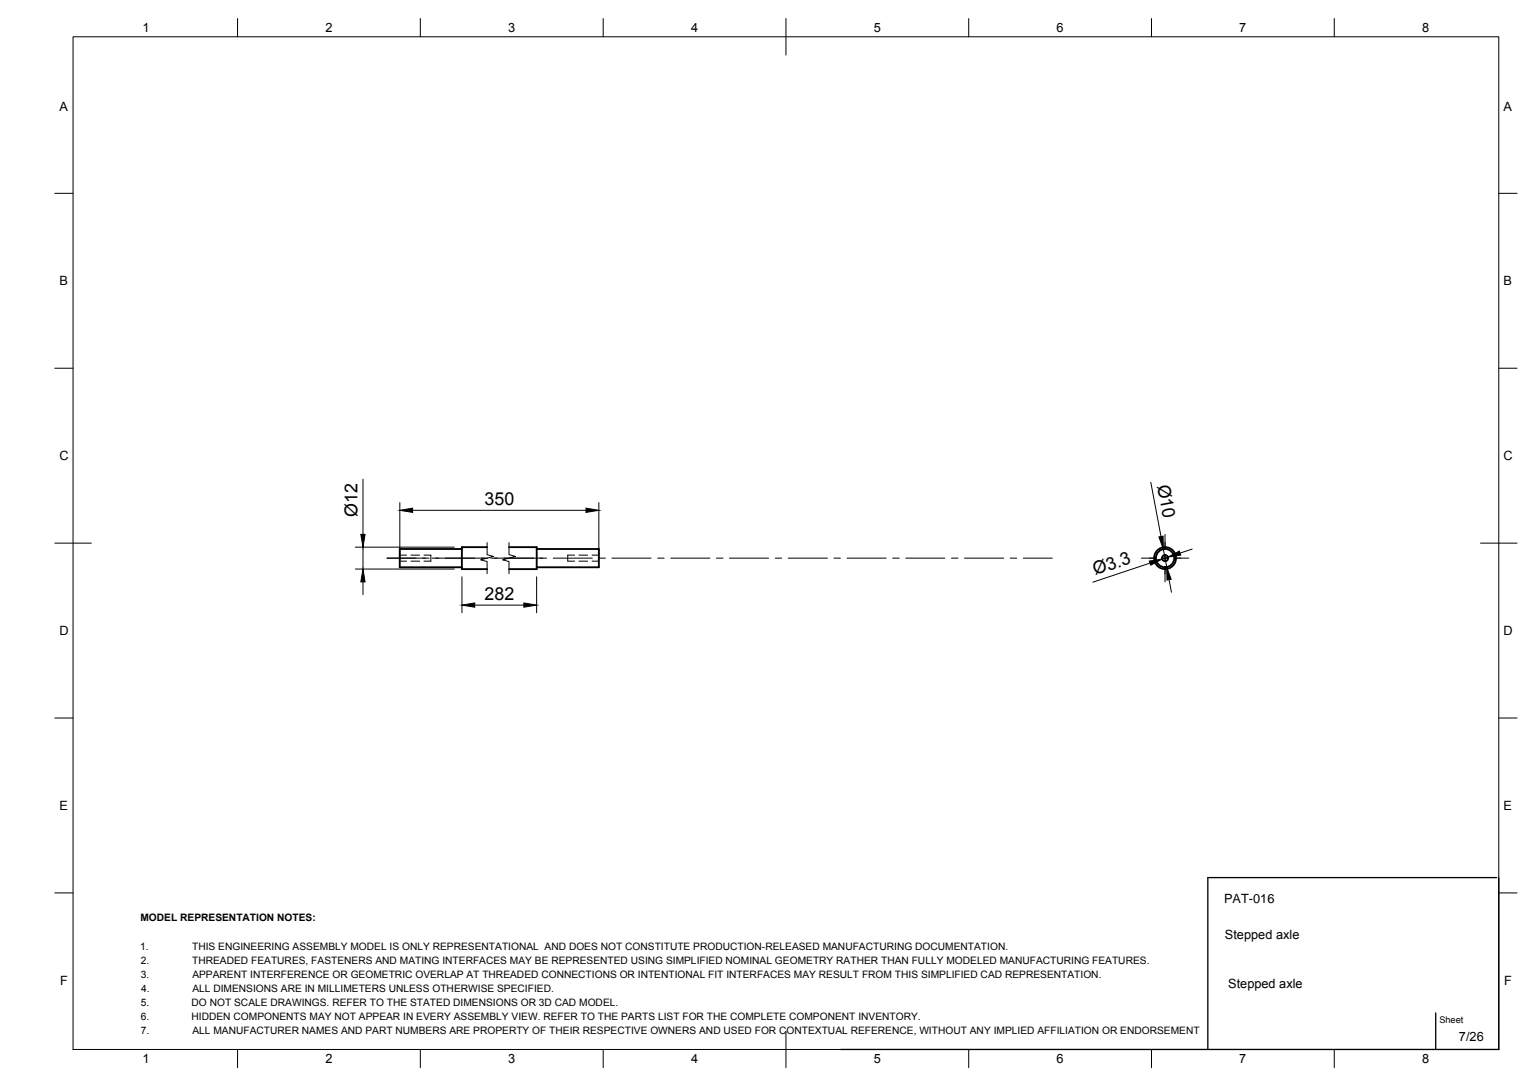
ISO-10303-21;
HEADER;
/* Generated by software containing ST-Developer
 * from STEP Tools, Inc. (www.steptools.com) 
 */

FILE_DESCRIPTION(
/* description */ ('Bracket-mounted idler roller'),
/* implementation_level */ '2;1');

FILE_NAME(
/* name */ 'Stepped axle.step',
/* time_stamp */ '2026-10-28T03:26:42-07:00',
/* author */ (''),
/* organization */ (''),
/* preprocessor_version */ 'ST-DEVELOPER v20.2',
/* originating_system */ 'Autodesk Translation Framework v15.17.0.0',
/* authorisation */ '');

FILE_SCHEMA (('AUTOMOTIVE_DESIGN { 1 0 10303 214 3 1 1 }'));
ENDSEC;

DATA;
#10=MECHANICAL_DESIGN_GEOMETRIC_PRESENTATION_REPRESENTATION('',(#282),#6241);
#240=SHAPE_REPRESENTATION_RELATIONSHIP('SRR','None',#6344,#261);
#261=ADVANCED_BREP_SHAPE_REPRESENTATION('',(#311),#6220);
#282=STYLED_ITEM('',(#6538),#311);
#311=MANIFOLD_SOLID_BREP('Body1',#3184);
#350=FACE_BOUND('',#754,.T.);
#351=FACE_BOUND('',#756,.T.);
#352=FACE_BOUND('',#761,.T.);
#353=FACE_BOUND('',#763,.T.);
#439=PLANE('',#3493);
#440=PLANE('',#3497);
#441=PLANE('',#3498);
#442=PLANE('',#3501);
#443=PLANE('',#3509);
#444=PLANE('',#3510);
#544=FACE_OUTER_BOUND('',#749,.T.);
#545=FACE_OUTER_BOUND('',#750,.T.);
#546=FACE_OUTER_BOUND('',#751,.T.);
#547=FACE_OUTER_BOUND('',#752,.T.);
#548=FACE_OUTER_BOUND('',#753,.T.);
#549=FACE_OUTER_BOUND('',#755,.T.);
#550=FACE_OUTER_BOUND('',#757,.T.);
#551=FACE_OUTER_BOUND('',#758,.T.);
#552=FACE_OUTER_BOUND('',#759,.T.);
#553=FACE_OUTER_BOUND('',#760,.T.);
#554=FACE_OUTER_BOUND('',#762,.T.);
#749=EDGE_LOOP('',(#2298,#2299,#2300,#2301));
#750=EDGE_LOOP('',(#2302));
#751=EDGE_LOOP('',(#2303,#2304,#2305,#2306));
#752=EDGE_LOOP('',(#2307));
#753=EDGE_LOOP('',(#2308));
#754=EDGE_LOOP('',(#2309));
#755=EDGE_LOOP('',(#2310));
#756=EDGE_LOOP('',(#2311));
#757=EDGE_LOOP('',(#2312,#2313,#2314,#2315));
#758=EDGE_LOOP('',(#2316,#2317,#2318,#2319));
#759=EDGE_LOOP('',(#2320,#2321,#2322,#2323));
#760=EDGE_LOOP('',(#2324));
#761=EDGE_LOOP('',(#2325));
#762=EDGE_LOOP('',(#2326));
#763=EDGE_LOOP('',(#2327));
#1033=LINE('',#5097,#1215);
#1034=LINE('',#5104,#1216);
#1035=LINE('',#5118,#1217);
#1036=LINE('',#5121,#1218);
#1037=LINE('',#5126,#1219);
#1215=VECTOR('',#4034,0.165);
#1216=VECTOR('',#4043,0.165);
#1217=VECTOR('',#4062,0.6);
#1218=VECTOR('',#4065,0.5);
#1219=VECTOR('',#4072,0.5);
#1355=CIRCLE('',#3491,0.165);
#1356=CIRCLE('',#3492,0.165);
#1357=CIRCLE('',#3495,0.165);
#1358=CIRCLE('',#3496,0.165);
#1359=CIRCLE('',#3499,0.6);
#1360=CIRCLE('',#3500,0.5);
#1361=CIRCLE('',#3502,0.6);
#1362=CIRCLE('',#3503,0.5);
#1363=CIRCLE('',#3506,0.5);
#1364=CIRCLE('',#3508,0.5);
#1568=VERTEX_POINT('',#5094);
#1569=VERTEX_POINT('',#5096);
#1570=VERTEX_POINT('',#5101);
#1571=VERTEX_POINT('',#5103);
#1572=VERTEX_POINT('',#5108);
#1573=VERTEX_POINT('',#5110);
#1574=VERTEX_POINT('',#5113);
#1575=VERTEX_POINT('',#5115);
#1576=VERTEX_POINT('',#5120);
#1577=VERTEX_POINT('',#5124);
#1851=EDGE_CURVE('',#1568,#1568,#1355,.T.);
#1852=EDGE_CURVE('',#1568,#1569,#1033,.T.);
#1853=EDGE_CURVE('',#1569,#1569,#1356,.T.);
#1854=EDGE_CURVE('',#1570,#1570,#1357,.T.);
#1855=EDGE_CURVE('',#1570,#1571,#1034,.T.);
#1856=EDGE_CURVE('',#1571,#1571,#1358,.T.);
#1857=EDGE_CURVE('',#1572,#1572,#1359,.T.);
#1858=EDGE_CURVE('',#1573,#1573,#1360,.T.);
#1859=EDGE_CURVE('',#1574,#1574,#1361,.T.);
#1860=EDGE_CURVE('',#1575,#1575,#1362,.T.);
#1861=EDGE_CURVE('',#1572,#1574,#1035,.T.);
#1862=EDGE_CURVE('',#1575,#1576,#1036,.T.);
#1863=EDGE_CURVE('',#1576,#1576,#1363,.T.);
#1864=EDGE_CURVE('',#1577,#1577,#1364,.T.);
#1865=EDGE_CURVE('',#1577,#1573,#1037,.T.);
#2298=ORIENTED_EDGE('',*,*,#1851,.F.);
#2299=ORIENTED_EDGE('',*,*,#1852,.T.);
#2300=ORIENTED_EDGE('',*,*,#1853,.F.);
#2301=ORIENTED_EDGE('',*,*,#1852,.F.);
#2302=ORIENTED_EDGE('',*,*,#1851,.T.);
#2303=ORIENTED_EDGE('',*,*,#1854,.F.);
#2304=ORIENTED_EDGE('',*,*,#1855,.T.);
#2305=ORIENTED_EDGE('',*,*,#1856,.T.);
#2306=ORIENTED_EDGE('',*,*,#1855,.F.);
#2307=ORIENTED_EDGE('',*,*,#1856,.F.);
#2308=ORIENTED_EDGE('',*,*,#1857,.T.);
#2309=ORIENTED_EDGE('',*,*,#1858,.F.);
#2310=ORIENTED_EDGE('',*,*,#1859,.F.);
#2311=ORIENTED_EDGE('',*,*,#1860,.F.);
#2312=ORIENTED_EDGE('',*,*,#1857,.F.);
#2313=ORIENTED_EDGE('',*,*,#1861,.T.);
#2314=ORIENTED_EDGE('',*,*,#1859,.T.);
#2315=ORIENTED_EDGE('',*,*,#1861,.F.);
#2316=ORIENTED_EDGE('',*,*,#1860,.T.);
#2317=ORIENTED_EDGE('',*,*,#1862,.T.);
#2318=ORIENTED_EDGE('',*,*,#1863,.T.);
#2319=ORIENTED_EDGE('',*,*,#1862,.F.);
#2320=ORIENTED_EDGE('',*,*,#1864,.F.);
#2321=ORIENTED_EDGE('',*,*,#1865,.T.);
#2322=ORIENTED_EDGE('',*,*,#1858,.T.);
#2323=ORIENTED_EDGE('',*,*,#1865,.F.);
#2324=ORIENTED_EDGE('',*,*,#1864,.T.);
#2325=ORIENTED_EDGE('',*,*,#1853,.T.);
#2326=ORIENTED_EDGE('',*,*,#1863,.F.);
#2327=ORIENTED_EDGE('',*,*,#1854,.T.);
#2934=CYLINDRICAL_SURFACE('',#3490,0.165);
#2935=CYLINDRICAL_SURFACE('',#3494,0.165);
#2936=CYLINDRICAL_SURFACE('',#3504,0.6);
#2937=CYLINDRICAL_SURFACE('',#3505,0.5);
#2938=CYLINDRICAL_SURFACE('',#3507,0.5);
#3019=ADVANCED_FACE('',(#544),#2934,.F.);
#3020=ADVANCED_FACE('',(#545),#439,.T.);
#3021=ADVANCED_FACE('',(#546),#2935,.F.);
#3022=ADVANCED_FACE('',(#547),#440,.F.);
#3023=ADVANCED_FACE('',(#548,#350),#441,.T.);
#3024=ADVANCED_FACE('',(#549,#351),#442,.F.);
#3025=ADVANCED_FACE('',(#550),#2936,.T.);
#3026=ADVANCED_FACE('',(#551),#2937,.T.);
#3027=ADVANCED_FACE('',(#552),#2938,.T.);
#3028=ADVANCED_FACE('',(#553,#352),#443,.T.);
#3029=ADVANCED_FACE('',(#554,#353),#444,.F.);
#3184=CLOSED_SHELL('',(#3019,#3020,#3021,#3022,#3023,#3024,#3025,#3026,
#3027,#3028,#3029));
#3489=AXIS2_PLACEMENT_3D('',#5092,#4028,#4029);
#3490=AXIS2_PLACEMENT_3D('',#5093,#4030,#4031);
#3491=AXIS2_PLACEMENT_3D('',#5095,#4032,#4033);
#3492=AXIS2_PLACEMENT_3D('',#5098,#4035,#4036);
#3493=AXIS2_PLACEMENT_3D('',#5099,#4037,#4038);
#3494=AXIS2_PLACEMENT_3D('',#5100,#4039,#4040);
#3495=AXIS2_PLACEMENT_3D('',#5102,#4041,#4042);
#3496=AXIS2_PLACEMENT_3D('',#5105,#4044,#4045);
#3497=AXIS2_PLACEMENT_3D('',#5106,#4046,#4047);
#3498=AXIS2_PLACEMENT_3D('',#5107,#4048,#4049);
#3499=AXIS2_PLACEMENT_3D('',#5109,#4050,#4051);
#3500=AXIS2_PLACEMENT_3D('',#5111,#4052,#4053);
#3501=AXIS2_PLACEMENT_3D('',#5112,#4054,#4055);
#3502=AXIS2_PLACEMENT_3D('',#5114,#4056,#4057);
#3503=AXIS2_PLACEMENT_3D('',#5116,#4058,#4059);
#3504=AXIS2_PLACEMENT_3D('',#5117,#4060,#4061);
#3505=AXIS2_PLACEMENT_3D('',#5119,#4063,#4064);
#3506=AXIS2_PLACEMENT_3D('',#5122,#4066,#4067);
#3507=AXIS2_PLACEMENT_3D('',#5123,#4068,#4069);
#3508=AXIS2_PLACEMENT_3D('',#5125,#4070,#4071);
#3509=AXIS2_PLACEMENT_3D('',#5127,#4073,#4074);
#3510=AXIS2_PLACEMENT_3D('',#5128,#4075,#4076);
#4028=DIRECTION('axis',(0.,0.,1.));
#4029=DIRECTION('refdir',(1.,0.,0.));
#4030=DIRECTION('center_axis',(0.,1.,0.));
#4031=DIRECTION('ref_axis',(1.,0.,0.));
#4032=DIRECTION('center_axis',(0.,1.,0.));
#4033=DIRECTION('ref_axis',(1.,0.,0.));
#4034=DIRECTION('',(0.,1.,0.));
#4035=DIRECTION('center_axis',(0.,-1.,0.));
#4036=DIRECTION('ref_axis',(1.,0.,0.));
#4037=DIRECTION('center_axis',(0.,1.,0.));
#4038=DIRECTION('ref_axis',(1.,0.,0.));
#4039=DIRECTION('center_axis',(0.,1.,0.));
#4040=DIRECTION('ref_axis',(1.,0.,0.));
#4041=DIRECTION('center_axis',(0.,1.,0.));
#4042=DIRECTION('ref_axis',(1.,0.,0.));
#4043=DIRECTION('',(0.,1.,0.));
#4044=DIRECTION('center_axis',(0.,1.,0.));
#4045=DIRECTION('ref_axis',(1.,0.,0.));
#4046=DIRECTION('center_axis',(0.,1.,0.));
#4047=DIRECTION('ref_axis',(1.,0.,0.));
#4048=DIRECTION('center_axis',(0.,1.,0.));
#4049=DIRECTION('ref_axis',(1.,0.,0.));
#4050=DIRECTION('center_axis',(0.,1.,0.));
#4051=DIRECTION('ref_axis',(1.,0.,0.));
#4052=DIRECTION('center_axis',(0.,1.,0.));
#4053=DIRECTION('ref_axis',(1.,0.,0.));
#4054=DIRECTION('center_axis',(0.,1.,0.));
#4055=DIRECTION('ref_axis',(1.,0.,0.));
#4056=DIRECTION('center_axis',(0.,1.,0.));
#4057=DIRECTION('ref_axis',(1.,0.,0.));
#4058=DIRECTION('center_axis',(0.,-1.,0.));
#4059=DIRECTION('ref_axis',(1.,0.,0.));
#4060=DIRECTION('center_axis',(0.,1.,0.));
#4061=DIRECTION('ref_axis',(1.,0.,0.));
#4062=DIRECTION('',(0.,-1.,0.));
#4063=DIRECTION('center_axis',(0.,1.,0.));
#4064=DIRECTION('ref_axis',(1.,0.,0.));
#4065=DIRECTION('',(0.,-1.,0.));
#4066=DIRECTION('center_axis',(0.,1.,0.));
#4067=DIRECTION('ref_axis',(1.,0.,0.));
#4068=DIRECTION('center_axis',(0.,1.,0.));
#4069=DIRECTION('ref_axis',(1.,0.,0.));
#4070=DIRECTION('center_axis',(0.,1.,0.));
#4071=DIRECTION('ref_axis',(1.,0.,0.));
#4072=DIRECTION('',(0.,-1.,0.));
#4073=DIRECTION('center_axis',(0.,1.,0.));
#4074=DIRECTION('ref_axis',(1.,0.,0.));
#4075=DIRECTION('center_axis',(0.,1.,0.));
#4076=DIRECTION('ref_axis',(1.,0.,0.));
#5092=CARTESIAN_POINT('',(0.,0.,0.));
#5093=CARTESIAN_POINT('Origin',(0.,30.8,4.5));
#5094=CARTESIAN_POINT('',(-0.165,30.8,4.5));
#5095=CARTESIAN_POINT('Origin',(0.,30.8,4.5));
#5096=CARTESIAN_POINT('',(-0.165,32.5,4.5));
#5097=CARTESIAN_POINT('',(-0.165,30.8,4.5));
#5098=CARTESIAN_POINT('Origin',(0.,32.5,4.5));
#5099=CARTESIAN_POINT('Origin',(0.,30.8,4.5));
#5100=CARTESIAN_POINT('Origin',(0.,-2.6,4.5));
#5101=CARTESIAN_POINT('',(-0.165,-2.5,4.5));
#5102=CARTESIAN_POINT('Origin',(0.,-2.5,4.5));
#5103=CARTESIAN_POINT('',(-0.165,-0.8,4.5));
#5104=CARTESIAN_POINT('',(-0.165,-2.6,4.5));
#5105=CARTESIAN_POINT('Origin',(0.,-0.8,4.5));
#5106=CARTESIAN_POINT('Origin',(0.,-0.8,4.5));
#5107=CARTESIAN_POINT('Origin',(0.,29.1,4.5));
#5108=CARTESIAN_POINT('',(-0.6,29.1,4.5));
#5109=CARTESIAN_POINT('Origin',(0.,29.1,4.5));
#5110=CARTESIAN_POINT('',(-0.5,29.1,4.5));
#5111=CARTESIAN_POINT('Origin',(0.,29.1,4.5));
#5112=CARTESIAN_POINT('Origin',(0.,0.9,4.5));
#5113=CARTESIAN_POINT('',(-0.6,0.9,4.5));
#5114=CARTESIAN_POINT('Origin',(0.,0.9,4.5));
#5115=CARTESIAN_POINT('',(-0.5,0.9,4.5));
#5116=CARTESIAN_POINT('Origin',(0.,0.9,4.5));
#5117=CARTESIAN_POINT('Origin',(0.,0.9,4.5));
#5118=CARTESIAN_POINT('',(-0.6,0.9,4.5));
#5119=CARTESIAN_POINT('Origin',(0.,-2.5,4.5));
#5120=CARTESIAN_POINT('',(-0.5,-2.5,4.5));
#5121=CARTESIAN_POINT('',(-0.5,-2.5,4.5));
#5122=CARTESIAN_POINT('Origin',(0.,-2.5,4.5));
#5123=CARTESIAN_POINT('Origin',(0.,-2.5,4.5));
#5124=CARTESIAN_POINT('',(-0.5,32.5,4.5));
#5125=CARTESIAN_POINT('Origin',(0.,32.5,4.5));
#5126=CARTESIAN_POINT('',(-0.5,-2.5,4.5));
#5127=CARTESIAN_POINT('Origin',(0.,32.5,4.5));
#5128=CARTESIAN_POINT('Origin',(0.,-2.5,4.5));
#6194=UNCERTAINTY_MEASURE_WITH_UNIT(LENGTH_MEASURE(0.001),#6242,
'DISTANCE_ACCURACY_VALUE',
'Maximum model space distance between geometric entities at asserted c
onnectivities');
#6215=UNCERTAINTY_MEASURE_WITH_UNIT(LENGTH_MEASURE(0.001),#6242,
'DISTANCE_ACCURACY_VALUE',
'Maximum model space distance between geometric entities at asserted c
onnectivities');
#6220=(
GEOMETRIC_REPRESENTATION_CONTEXT(3)
GLOBAL_UNCERTAINTY_ASSIGNED_CONTEXT((#6194))
GLOBAL_UNIT_ASSIGNED_CONTEXT((#6242,#6244,#6245))
REPRESENTATION_CONTEXT('','3D')
);
#6241=(
GEOMETRIC_REPRESENTATION_CONTEXT(3)
GLOBAL_UNCERTAINTY_ASSIGNED_CONTEXT((#6215))
GLOBAL_UNIT_ASSIGNED_CONTEXT((#6242,#6244,#6245))
REPRESENTATION_CONTEXT('','3D')
);
#6242=(
LENGTH_UNIT()
NAMED_UNIT(*)
SI_UNIT(.CENTI.,.METRE.)
);
#6244=(
NAMED_UNIT(*)
PLANE_ANGLE_UNIT()
SI_UNIT($,.RADIAN.)
);
#6245=(
NAMED_UNIT(*)
SI_UNIT($,.STERADIAN.)
SOLID_ANGLE_UNIT()
);
#6250=SHAPE_DEFINITION_REPRESENTATION(#6275,#6344);
#6275=PRODUCT_DEFINITION_SHAPE('',$,#6370);
#6344=SHAPE_REPRESENTATION('',(#3489),#6220);
#6365=PRODUCT_DEFINITION_CONTEXT('part definition',#6442,'design');
#6370=PRODUCT_DEFINITION('Stepped axle','Stepped axle',#6395,#6365);
#6395=PRODUCT_DEFINITION_FORMATION('',$,#6448);
#6442=APPLICATION_CONTEXT(
'Core Data for Automotive Mechanical Design Process');
#6443=PRODUCT_CONTEXT('part definition',#6442,'mechanical');
#6448=PRODUCT('Stepped axle','Stepped axle','Stepped axle',(#6443));
#6532=COLOUR_RGB('Grey',0.48,0.52,0.57);
#6533=FILL_AREA_STYLE_COLOUR('',#6532);
#6534=FILL_AREA_STYLE('',(#6533));
#6535=SURFACE_STYLE_FILL_AREA(#6534);
#6536=SURFACE_SIDE_STYLE('',(#6535));
#6537=SURFACE_STYLE_USAGE(.BOTH.,#6536);
#6538=PRESENTATION_STYLE_ASSIGNMENT((#6537));
ENDSEC;
END-ISO-10303-21;
